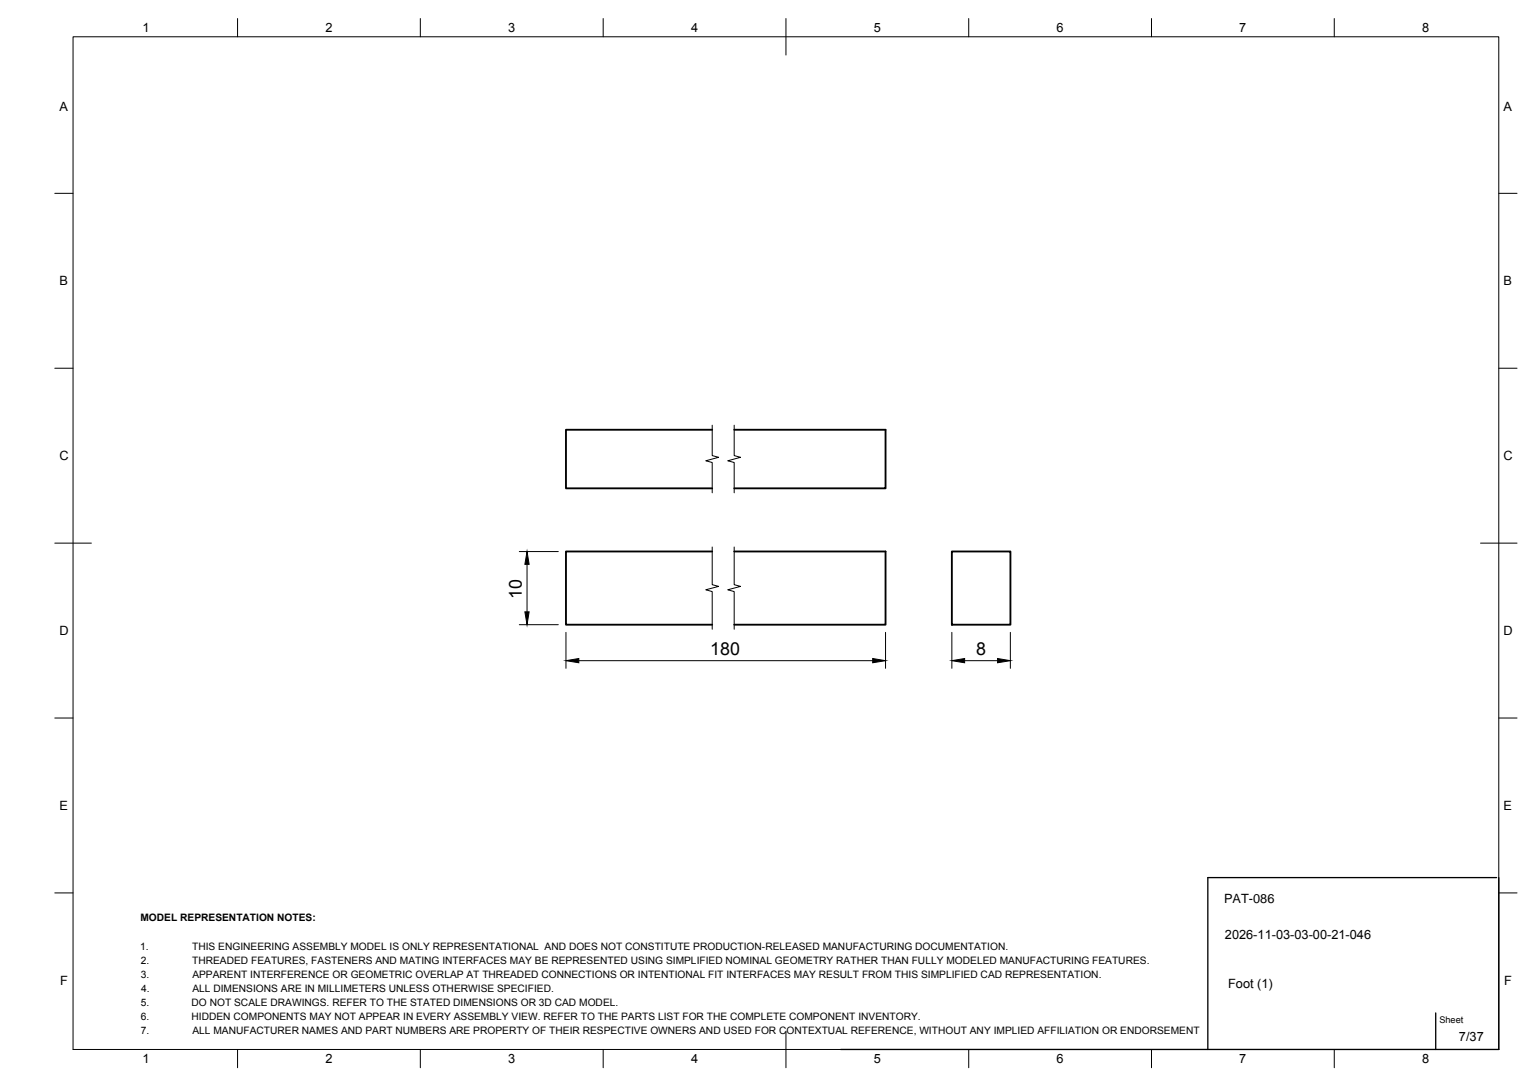
ISO-10303-21;
HEADER;
/* Generated by software containing ST-Developer
 * from STEP Tools, Inc. (www.steptools.com) 
 */

FILE_DESCRIPTION(
/* description */ ('Ratchet and pawl hand winch drum'),
/* implementation_level */ '2;1');

FILE_NAME(
/* name */ 'Foot (1).step',
/* time_stamp */ '2026-10-27T12:42:58-07:00',
/* author */ (''),
/* organization */ (''),
/* preprocessor_version */ 'ST-DEVELOPER v20.2',
/* originating_system */ 'Autodesk Translation Framework v15.17.0.0',
/* authorisation */ '');

FILE_SCHEMA (('AUTOMOTIVE_DESIGN { 1 0 10303 214 3 1 1 }'));
ENDSEC;

DATA;
#10=MECHANICAL_DESIGN_GEOMETRIC_PRESENTATION_REPRESENTATION('',(#391),#11801);
#323=SHAPE_REPRESENTATION_RELATIONSHIP('SRR','None',#11949,#357);
#357=ADVANCED_BREP_SHAPE_REPRESENTATION('',(#426),#11766);
#391=STYLED_ITEM('',(#12227),#426);
#426=MANIFOLD_SOLID_BREP('Body1',#6268);
#613=PLANE('',#6726);
#614=PLANE('',#6727);
#615=PLANE('',#6728);
#616=PLANE('',#6729);
#617=PLANE('',#6730);
#618=PLANE('',#6731);
#862=FACE_OUTER_BOUND('',#1238,.T.);
#863=FACE_OUTER_BOUND('',#1239,.T.);
#864=FACE_OUTER_BOUND('',#1240,.T.);
#865=FACE_OUTER_BOUND('',#1241,.T.);
#866=FACE_OUTER_BOUND('',#1242,.T.);
#867=FACE_OUTER_BOUND('',#1243,.T.);
#1238=EDGE_LOOP('',(#4355,#4356,#4357,#4358));
#1239=EDGE_LOOP('',(#4359,#4360,#4361,#4362));
#1240=EDGE_LOOP('',(#4363,#4364,#4365,#4366));
#1241=EDGE_LOOP('',(#4367,#4368,#4369,#4370));
#1242=EDGE_LOOP('',(#4371,#4372,#4373,#4374));
#1243=EDGE_LOOP('',(#4375,#4376,#4377,#4378));
#1731=LINE('',#9347,#2242);
#1732=LINE('',#9349,#2243);
#1733=LINE('',#9351,#2244);
#1734=LINE('',#9352,#2245);
#1735=LINE('',#9355,#2246);
#1736=LINE('',#9357,#2247);
#1737=LINE('',#9358,#2248);
#1738=LINE('',#9361,#2249);
#1739=LINE('',#9363,#2250);
#1740=LINE('',#9364,#2251);
#1741=LINE('',#9366,#2252);
#1742=LINE('',#9367,#2253);
#2242=VECTOR('',#7488,1.);
#2243=VECTOR('',#7489,1.);
#2244=VECTOR('',#7490,1.);
#2245=VECTOR('',#7491,1.);
#2246=VECTOR('',#7494,1.);
#2247=VECTOR('',#7495,1.);
#2248=VECTOR('',#7496,1.);
#2249=VECTOR('',#7499,1.);
#2250=VECTOR('',#7500,1.);
#2251=VECTOR('',#7501,1.);
#2252=VECTOR('',#7504,1.);
#2253=VECTOR('',#7505,1.);
#2978=VERTEX_POINT('',#9345);
#2979=VERTEX_POINT('',#9346);
#2980=VERTEX_POINT('',#9348);
#2981=VERTEX_POINT('',#9350);
#2982=VERTEX_POINT('',#9354);
#2983=VERTEX_POINT('',#9356);
#2984=VERTEX_POINT('',#9360);
#2985=VERTEX_POINT('',#9362);
#3521=EDGE_CURVE('',#2978,#2979,#1731,.T.);
#3522=EDGE_CURVE('',#2979,#2980,#1732,.T.);
#3523=EDGE_CURVE('',#2981,#2980,#1733,.T.);
#3524=EDGE_CURVE('',#2978,#2981,#1734,.T.);
#3525=EDGE_CURVE('',#2982,#2978,#1735,.T.);
#3526=EDGE_CURVE('',#2983,#2981,#1736,.T.);
#3527=EDGE_CURVE('',#2982,#2983,#1737,.T.);
#3528=EDGE_CURVE('',#2984,#2982,#1738,.T.);
#3529=EDGE_CURVE('',#2985,#2983,#1739,.T.);
#3530=EDGE_CURVE('',#2984,#2985,#1740,.T.);
#3531=EDGE_CURVE('',#2979,#2984,#1741,.T.);
#3532=EDGE_CURVE('',#2980,#2985,#1742,.T.);
#4355=ORIENTED_EDGE('',*,*,#3521,.T.);
#4356=ORIENTED_EDGE('',*,*,#3522,.T.);
#4357=ORIENTED_EDGE('',*,*,#3523,.F.);
#4358=ORIENTED_EDGE('',*,*,#3524,.F.);
#4359=ORIENTED_EDGE('',*,*,#3525,.T.);
#4360=ORIENTED_EDGE('',*,*,#3524,.T.);
#4361=ORIENTED_EDGE('',*,*,#3526,.F.);
#4362=ORIENTED_EDGE('',*,*,#3527,.F.);
#4363=ORIENTED_EDGE('',*,*,#3528,.T.);
#4364=ORIENTED_EDGE('',*,*,#3527,.T.);
#4365=ORIENTED_EDGE('',*,*,#3529,.F.);
#4366=ORIENTED_EDGE('',*,*,#3530,.F.);
#4367=ORIENTED_EDGE('',*,*,#3531,.T.);
#4368=ORIENTED_EDGE('',*,*,#3530,.T.);
#4369=ORIENTED_EDGE('',*,*,#3532,.F.);
#4370=ORIENTED_EDGE('',*,*,#3522,.F.);
#4371=ORIENTED_EDGE('',*,*,#3532,.T.);
#4372=ORIENTED_EDGE('',*,*,#3529,.T.);
#4373=ORIENTED_EDGE('',*,*,#3526,.T.);
#4374=ORIENTED_EDGE('',*,*,#3523,.T.);
#4375=ORIENTED_EDGE('',*,*,#3531,.F.);
#4376=ORIENTED_EDGE('',*,*,#3521,.F.);
#4377=ORIENTED_EDGE('',*,*,#3525,.F.);
#4378=ORIENTED_EDGE('',*,*,#3528,.F.);
#5932=ADVANCED_FACE('',(#862),#613,.T.);
#5933=ADVANCED_FACE('',(#863),#614,.T.);
#5934=ADVANCED_FACE('',(#864),#615,.T.);
#5935=ADVANCED_FACE('',(#865),#616,.T.);
#5936=ADVANCED_FACE('',(#866),#617,.T.);
#5937=ADVANCED_FACE('',(#867),#618,.F.);
#6268=CLOSED_SHELL('',(#5932,#5933,#5934,#5935,#5936,#5937));
#6725=AXIS2_PLACEMENT_3D('',#9343,#7484,#7485);
#6726=AXIS2_PLACEMENT_3D('',#9344,#7486,#7487);
#6727=AXIS2_PLACEMENT_3D('',#9353,#7492,#7493);
#6728=AXIS2_PLACEMENT_3D('',#9359,#7497,#7498);
#6729=AXIS2_PLACEMENT_3D('',#9365,#7502,#7503);
#6730=AXIS2_PLACEMENT_3D('',#9368,#7506,#7507);
#6731=AXIS2_PLACEMENT_3D('',#9369,#7508,#7509);
#7484=DIRECTION('axis',(0.,0.,1.));
#7485=DIRECTION('refdir',(1.,0.,0.));
#7486=DIRECTION('center_axis',(0.,1.,0.));
#7487=DIRECTION('ref_axis',(-1.,0.,0.));
#7488=DIRECTION('',(-1.,0.,0.));
#7489=DIRECTION('',(0.,0.,1.));
#7490=DIRECTION('',(-1.,0.,0.));
#7491=DIRECTION('',(0.,0.,1.));
#7492=DIRECTION('center_axis',(1.,0.,0.));
#7493=DIRECTION('ref_axis',(0.,1.,0.));
#7494=DIRECTION('',(0.,1.,0.));
#7495=DIRECTION('',(0.,1.,0.));
#7496=DIRECTION('',(0.,0.,1.));
#7497=DIRECTION('center_axis',(0.,-1.,0.));
#7498=DIRECTION('ref_axis',(1.,0.,0.));
#7499=DIRECTION('',(1.,0.,0.));
#7500=DIRECTION('',(1.,0.,0.));
#7501=DIRECTION('',(0.,0.,1.));
#7502=DIRECTION('center_axis',(-1.,0.,0.));
#7503=DIRECTION('ref_axis',(0.,-1.,0.));
#7504=DIRECTION('',(0.,-1.,0.));
#7505=DIRECTION('',(0.,-1.,0.));
#7506=DIRECTION('center_axis',(0.,0.,1.));
#7507=DIRECTION('ref_axis',(1.,0.,0.));
#7508=DIRECTION('center_axis',(0.,0.,1.));
#7509=DIRECTION('ref_axis',(1.,0.,0.));
#9343=CARTESIAN_POINT('',(0.,0.,0.));
#9344=CARTESIAN_POINT('Origin',(10.,20.5,-0.8));
#9345=CARTESIAN_POINT('',(10.,20.5,-0.8));
#9346=CARTESIAN_POINT('',(-8.,20.5,-0.8));
#9347=CARTESIAN_POINT('',(10.,20.5,-0.8));
#9348=CARTESIAN_POINT('',(-8.,20.5,0.));
#9349=CARTESIAN_POINT('',(-8.,20.5,-0.8));
#9350=CARTESIAN_POINT('',(10.,20.5,0.));
#9351=CARTESIAN_POINT('',(10.,20.5,0.));
#9352=CARTESIAN_POINT('',(10.,20.5,-0.8));
#9353=CARTESIAN_POINT('Origin',(10.,19.5,-0.8));
#9354=CARTESIAN_POINT('',(10.,19.5,-0.8));
#9355=CARTESIAN_POINT('',(10.,19.5,-0.8));
#9356=CARTESIAN_POINT('',(10.,19.5,0.));
#9357=CARTESIAN_POINT('',(10.,19.5,0.));
#9358=CARTESIAN_POINT('',(10.,19.5,-0.8));
#9359=CARTESIAN_POINT('Origin',(-8.,19.5,-0.8));
#9360=CARTESIAN_POINT('',(-8.,19.5,-0.8));
#9361=CARTESIAN_POINT('',(-8.,19.5,-0.8));
#9362=CARTESIAN_POINT('',(-8.,19.5,0.));
#9363=CARTESIAN_POINT('',(-8.,19.5,0.));
#9364=CARTESIAN_POINT('',(-8.,19.5,-0.8));
#9365=CARTESIAN_POINT('Origin',(-8.,20.5,-0.8));
#9366=CARTESIAN_POINT('',(-8.,20.5,-0.8));
#9367=CARTESIAN_POINT('',(-8.,20.5,0.));
#9368=CARTESIAN_POINT('Origin',(1.,20.,0.));
#9369=CARTESIAN_POINT('Origin',(1.,20.,-0.8));
#11726=UNCERTAINTY_MEASURE_WITH_UNIT(LENGTH_MEASURE(0.001),#11802,
'DISTANCE_ACCURACY_VALUE',
'Maximum model space distance between geometric entities at asserted c
onnectivities');
#11761=UNCERTAINTY_MEASURE_WITH_UNIT(LENGTH_MEASURE(0.001),#11802,
'DISTANCE_ACCURACY_VALUE',
'Maximum model space distance between geometric entities at asserted c
onnectivities');
#11766=(
GEOMETRIC_REPRESENTATION_CONTEXT(3)
GLOBAL_UNCERTAINTY_ASSIGNED_CONTEXT((#11726))
GLOBAL_UNIT_ASSIGNED_CONTEXT((#11802,#11804,#11805))
REPRESENTATION_CONTEXT('','3D')
);
#11801=(
GEOMETRIC_REPRESENTATION_CONTEXT(3)
GLOBAL_UNCERTAINTY_ASSIGNED_CONTEXT((#11761))
GLOBAL_UNIT_ASSIGNED_CONTEXT((#11802,#11804,#11805))
REPRESENTATION_CONTEXT('','3D')
);
#11802=(
LENGTH_UNIT()
NAMED_UNIT(*)
SI_UNIT(.CENTI.,.METRE.)
);
#11804=(
NAMED_UNIT(*)
PLANE_ANGLE_UNIT()
SI_UNIT($,.RADIAN.)
);
#11805=(
NAMED_UNIT(*)
SI_UNIT($,.STERADIAN.)
SOLID_ANGLE_UNIT()
);
#11810=SHAPE_DEFINITION_REPRESENTATION(#11849,#11949);
#11849=PRODUCT_DEFINITION_SHAPE('',$,#11989);
#11949=SHAPE_REPRESENTATION('',(#6725),#11766);
#11984=PRODUCT_DEFINITION_CONTEXT('part definition',#12103,'design');
#11989=PRODUCT_DEFINITION('Foot (1)','Foot (1)',#12028,#11984);
#12028=PRODUCT_DEFINITION_FORMATION('',$,#12109);
#12103=APPLICATION_CONTEXT(
'Core Data for Automotive Mechanical Design Process');
#12104=PRODUCT_CONTEXT('part definition',#12103,'mechanical');
#12109=PRODUCT('Foot (1)','Foot (1)','Foot (1)',(#12104));
#12221=COLOUR_RGB('Off White',0.89,0.88,0.83);
#12222=FILL_AREA_STYLE_COLOUR('',#12221);
#12223=FILL_AREA_STYLE('',(#12222));
#12224=SURFACE_STYLE_FILL_AREA(#12223);
#12225=SURFACE_SIDE_STYLE('',(#12224));
#12226=SURFACE_STYLE_USAGE(.BOTH.,#12225);
#12227=PRESENTATION_STYLE_ASSIGNMENT((#12226));
ENDSEC;
END-ISO-10303-21;
